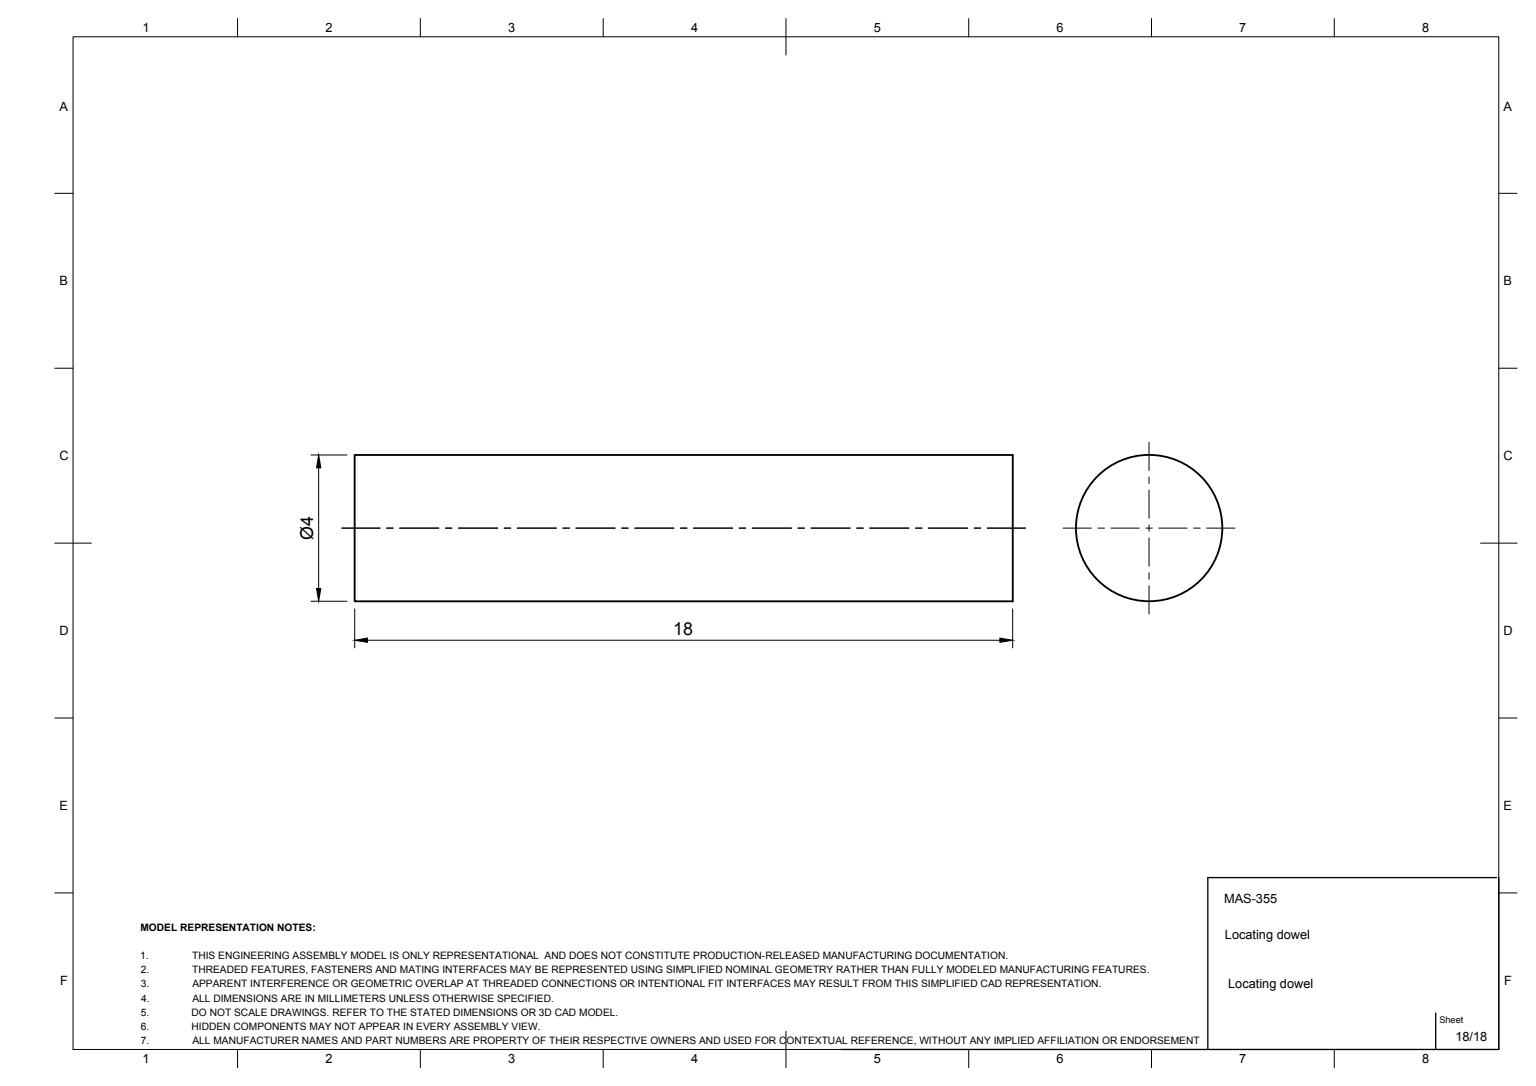
ISO-10303-21;
HEADER;
/* Generated by software containing ST-Developer
 * from STEP Tools, Inc. (www.steptools.com) 
 */

FILE_DESCRIPTION(
/* description */ ('Independent two-stage fixed-ring planetary gearbox,24/24/72 teeth,mod
ule2,20deg involutes,three planets per stage,4:1 x4:1=16:1. Native cut
-space/fillet/pattern tooth profiles derived from reusable gear blanks
; shared sun/planet/ring/carrier parts across both stages. Captured br
onze-journal input/carriers, headed retained planet pins, keyed inters
tage drive and modular keyed output interface. Native ideal gear links
; no torque, precision grade, production backlash/fits, lubrication, s
peed or life rating.'),
/* implementation_level */ '2;1');

FILE_NAME(
/* name */ 'Locating dowel.step',
/* time_stamp */ '2026-11-08T19:10:00-08:00',
/* author */ (''),
/* organization */ (''),
/* preprocessor_version */ 'ST-DEVELOPER v20.2',
/* originating_system */ 'Autodesk Translation Framework v15.17.0.0',
/* authorisation */ '');

FILE_SCHEMA (('AUTOMOTIVE_DESIGN { 1 0 10303 214 3 1 1 }'));
ENDSEC;

DATA;
#10=MECHANICAL_DESIGN_GEOMETRIC_PRESENTATION_REPRESENTATION('',(#1181),#259224);
#1141=SHAPE_REPRESENTATION_RELATIONSHIP('SRR','None',#259388,#1161);
#1161=ADVANCED_BREP_SHAPE_REPRESENTATION('',(#1201),#259222);
#1181=STYLED_ITEM('',(#259491),#1201);
#1201=MANIFOLD_SOLID_BREP('Body1',#25168);
#1686=PLANE('',#27174);
#1687=PLANE('',#27175);
#2986=FACE_OUTER_BOUND('',#4445,.T.);
#2987=FACE_OUTER_BOUND('',#4446,.T.);
#2988=FACE_OUTER_BOUND('',#4447,.T.);
#4445=EDGE_LOOP('',(#22766,#22767,#22768,#22769));
#4446=EDGE_LOOP('',(#22770));
#4447=EDGE_LOOP('',(#22771));
#5377=CIRCLE('',#27172,2.);
#5378=CIRCLE('',#27173,2.);
#7792=LINE('',#256104,#8977);
#8977=VECTOR('',#32023,2.);
#11493=VERTEX_POINT('',#256101);
#11494=VERTEX_POINT('',#256103);
#15268=EDGE_CURVE('',#11493,#11493,#5377,.T.);
#15269=EDGE_CURVE('',#11493,#11494,#7792,.T.);
#15270=EDGE_CURVE('',#11494,#11494,#5378,.T.);
#22766=ORIENTED_EDGE('',*,*,#15268,.F.);
#22767=ORIENTED_EDGE('',*,*,#15269,.T.);
#22768=ORIENTED_EDGE('',*,*,#15270,.T.);
#22769=ORIENTED_EDGE('',*,*,#15269,.F.);
#22770=ORIENTED_EDGE('',*,*,#15268,.T.);
#22771=ORIENTED_EDGE('',*,*,#15270,.F.);
#23760=CYLINDRICAL_SURFACE('',#27171,2.);
#25092=ADVANCED_FACE('',(#2986),#23760,.T.);
#25093=ADVANCED_FACE('',(#2987),#1686,.T.);
#25094=ADVANCED_FACE('',(#2988),#1687,.F.);
#25168=CLOSED_SHELL('',(#25092,#25093,#25094));
#27170=AXIS2_PLACEMENT_3D('',#256099,#32017,#32018);
#27171=AXIS2_PLACEMENT_3D('',#256100,#32019,#32020);
#27172=AXIS2_PLACEMENT_3D('',#256102,#32021,#32022);
#27173=AXIS2_PLACEMENT_3D('',#256105,#32024,#32025);
#27174=AXIS2_PLACEMENT_3D('',#256106,#32026,#32027);
#27175=AXIS2_PLACEMENT_3D('',#256107,#32028,#32029);
#32017=DIRECTION('axis',(0.,0.,1.));
#32018=DIRECTION('refdir',(1.,0.,0.));
#32019=DIRECTION('center_axis',(0.,0.,1.));
#32020=DIRECTION('ref_axis',(1.,0.,0.));
#32021=DIRECTION('center_axis',(0.,0.,1.));
#32022=DIRECTION('ref_axis',(1.,0.,0.));
#32023=DIRECTION('',(0.,0.,-1.));
#32024=DIRECTION('center_axis',(0.,0.,1.));
#32025=DIRECTION('ref_axis',(1.,0.,0.));
#32026=DIRECTION('center_axis',(0.,0.,1.));
#32027=DIRECTION('ref_axis',(1.,0.,0.));
#32028=DIRECTION('center_axis',(0.,0.,1.));
#32029=DIRECTION('ref_axis',(1.,0.,0.));
#256099=CARTESIAN_POINT('',(0.,0.,0.));
#256100=CARTESIAN_POINT('Origin',(0.,0.,0.));
#256101=CARTESIAN_POINT('',(-2.,-2.44929359829471E-16,18.));
#256102=CARTESIAN_POINT('Origin',(0.,0.,18.));
#256103=CARTESIAN_POINT('',(-2.,-2.44929359829471E-16,0.));
#256104=CARTESIAN_POINT('',(-2.,-2.44929359829471E-16,0.));
#256105=CARTESIAN_POINT('Origin',(0.,0.,0.));
#256106=CARTESIAN_POINT('Origin',(0.,0.,18.));
#256107=CARTESIAN_POINT('Origin',(0.,0.,0.));
#259200=UNCERTAINTY_MEASURE_WITH_UNIT(LENGTH_MEASURE(0.01),#259225,
'DISTANCE_ACCURACY_VALUE',
'Maximum model space distance between geometric entities at asserted c
onnectivities');
#259202=UNCERTAINTY_MEASURE_WITH_UNIT(LENGTH_MEASURE(0.01),#259225,
'DISTANCE_ACCURACY_VALUE',
'Maximum model space distance between geometric entities at asserted c
onnectivities');
#259222=(
GEOMETRIC_REPRESENTATION_CONTEXT(3)
GLOBAL_UNCERTAINTY_ASSIGNED_CONTEXT((#259200))
GLOBAL_UNIT_ASSIGNED_CONTEXT((#259225,#259227,#259228))
REPRESENTATION_CONTEXT('','3D')
);
#259224=(
GEOMETRIC_REPRESENTATION_CONTEXT(3)
GLOBAL_UNCERTAINTY_ASSIGNED_CONTEXT((#259202))
GLOBAL_UNIT_ASSIGNED_CONTEXT((#259225,#259227,#259228))
REPRESENTATION_CONTEXT('','3D')
);
#259225=(
LENGTH_UNIT()
NAMED_UNIT(*)
SI_UNIT(.MILLI.,.METRE.)
);
#259227=(
NAMED_UNIT(*)
PLANE_ANGLE_UNIT()
SI_UNIT($,.RADIAN.)
);
#259228=(
NAMED_UNIT(*)
SI_UNIT($,.STERADIAN.)
SOLID_ANGLE_UNIT()
);
#259248=SHAPE_DEFINITION_REPRESENTATION(#259269,#259388);
#259269=PRODUCT_DEFINITION_SHAPE('',$,#259410);
#259388=SHAPE_REPRESENTATION('',(#27170),#259222);
#259390=PRODUCT_DEFINITION_CONTEXT('part definition',#259455,'design');
#259410=PRODUCT_DEFINITION('Locating dowel','Locating dowel',#259431,#259390);
#259431=PRODUCT_DEFINITION_FORMATION('',$,#259476);
#259455=APPLICATION_CONTEXT(
'Core Data for Automotive Mechanical Design Process');
#259456=PRODUCT_CONTEXT('part definition',#259455,'mechanical');
#259476=PRODUCT('Locating dowel','Locating dowel',$,(#259456));
#259491=PRESENTATION_STYLE_ASSIGNMENT((#259506));
#259506=SURFACE_STYLE_USAGE(.BOTH.,#259521);
#259521=SURFACE_SIDE_STYLE('',(#259536));
#259536=SURFACE_STYLE_FILL_AREA(#259551);
#259551=FILL_AREA_STYLE('Dowel gray',(#259566));
#259566=FILL_AREA_STYLE_COLOUR('Dowel gray',#259581);
#259581=COLOUR_RGB('Dowel gray',0.576470588235294,0.615686274509804,0.666666666666667);
ENDSEC;
END-ISO-10303-21;
